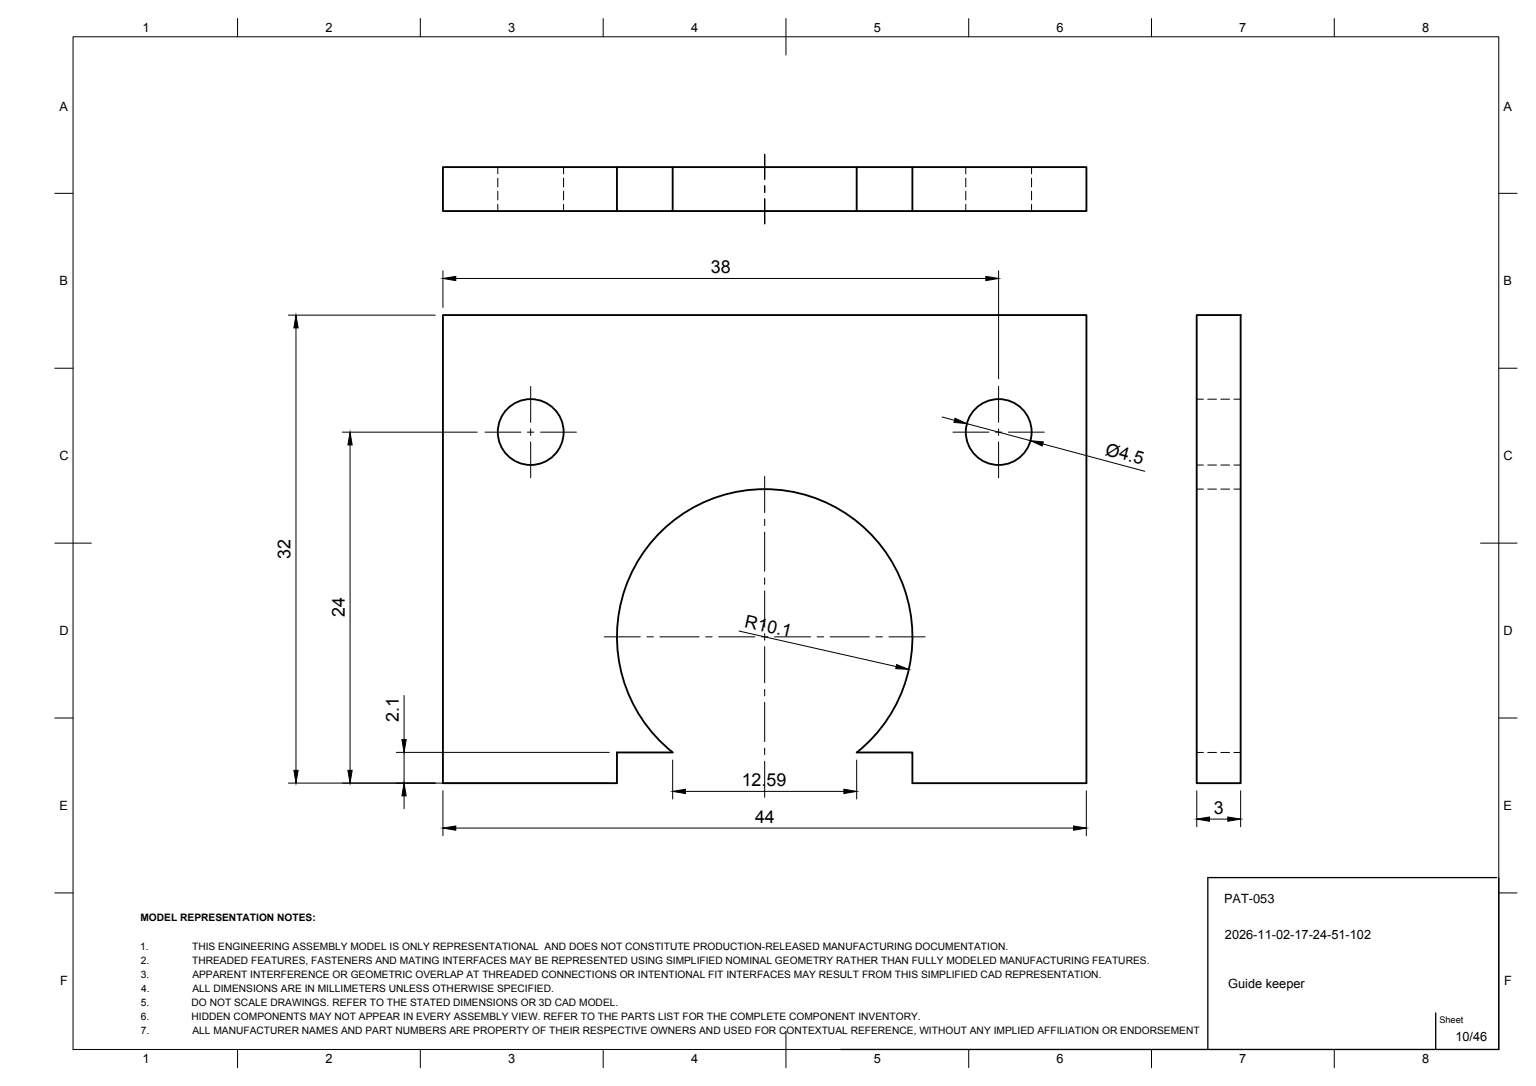
ISO-10303-21;
HEADER;
/* Generated by software containing ST-Developer
 * from STEP Tools, Inc. (www.steptools.com) 
 */

FILE_DESCRIPTION(
/* description */ ('Hand-operated arbor press'),
/* implementation_level */ '2;1');

FILE_NAME(
/* name */ 'Guide keeper.step',
/* time_stamp */ '2026-10-28T03:25:25-07:00',
/* author */ (''),
/* organization */ (''),
/* preprocessor_version */ 'ST-DEVELOPER v20.2',
/* originating_system */ 'Autodesk Translation Framework v15.17.0.0',
/* authorisation */ '');

FILE_SCHEMA (('AUTOMOTIVE_DESIGN { 1 0 10303 214 3 1 1 }'));
ENDSEC;

DATA;
#10=MECHANICAL_DESIGN_GEOMETRIC_PRESENTATION_REPRESENTATION('',(#591),#32751);
#507=SHAPE_REPRESENTATION_RELATIONSHIP('SRR','None',#32936,#549);
#549=ADVANCED_BREP_SHAPE_REPRESENTATION('',(#640),#32710);
#591=STYLED_ITEM('',(#33235),#640);
#640=MANIFOLD_SOLID_BREP('Body1',#12488);
#715=FACE_BOUND('',#2097,.T.);
#716=FACE_BOUND('',#2098,.T.);
#717=FACE_BOUND('',#2104,.T.);
#718=FACE_BOUND('',#2105,.T.);
#901=PLANE('',#13146);
#902=PLANE('',#13147);
#903=PLANE('',#13148);
#904=PLANE('',#13149);
#905=PLANE('',#13150);
#906=PLANE('',#13151);
#907=PLANE('',#13152);
#908=PLANE('',#13156);
#909=PLANE('',#13157);
#910=PLANE('',#13158);
#911=PLANE('',#13159);
#1372=FACE_OUTER_BOUND('',#2088,.T.);
#1373=FACE_OUTER_BOUND('',#2089,.T.);
#1374=FACE_OUTER_BOUND('',#2090,.T.);
#1375=FACE_OUTER_BOUND('',#2091,.T.);
#1376=FACE_OUTER_BOUND('',#2092,.T.);
#1377=FACE_OUTER_BOUND('',#2093,.T.);
#1378=FACE_OUTER_BOUND('',#2094,.T.);
#1379=FACE_OUTER_BOUND('',#2095,.T.);
#1380=FACE_OUTER_BOUND('',#2096,.T.);
#1381=FACE_OUTER_BOUND('',#2099,.T.);
#1382=FACE_OUTER_BOUND('',#2100,.T.);
#1383=FACE_OUTER_BOUND('',#2101,.T.);
#1384=FACE_OUTER_BOUND('',#2102,.T.);
#1385=FACE_OUTER_BOUND('',#2103,.T.);
#2088=EDGE_LOOP('',(#8696,#8697,#8698,#8699));
#2089=EDGE_LOOP('',(#8700,#8701,#8702,#8703));
#2090=EDGE_LOOP('',(#8704,#8705,#8706,#8707));
#2091=EDGE_LOOP('',(#8708,#8709,#8710,#8711));
#2092=EDGE_LOOP('',(#8712,#8713,#8714,#8715));
#2093=EDGE_LOOP('',(#8716,#8717,#8718,#8719));
#2094=EDGE_LOOP('',(#8720,#8721,#8722,#8723));
#2095=EDGE_LOOP('',(#8724,#8725,#8726,#8727));
#2096=EDGE_LOOP('',(#8728,#8729,#8730,#8731,#8732,#8733,#8734,#8735,#8736,
#8737));
#2097=EDGE_LOOP('',(#8738));
#2098=EDGE_LOOP('',(#8739));
#2099=EDGE_LOOP('',(#8740,#8741,#8742,#8743));
#2100=EDGE_LOOP('',(#8744,#8745,#8746,#8747));
#2101=EDGE_LOOP('',(#8748,#8749,#8750,#8751));
#2102=EDGE_LOOP('',(#8752,#8753,#8754,#8755));
#2103=EDGE_LOOP('',(#8756,#8757,#8758,#8759,#8760,#8761,#8762,#8763,#8764,
#8765));
#2104=EDGE_LOOP('',(#8766));
#2105=EDGE_LOOP('',(#8767));
#2956=LINE('',#18039,#4127);
#2957=LINE('',#18045,#4128);
#2958=LINE('',#18050,#4129);
#2959=LINE('',#18052,#4130);
#2960=LINE('',#18054,#4131);
#2961=LINE('',#18055,#4132);
#2962=LINE('',#18059,#4133);
#2963=LINE('',#18061,#4134);
#2964=LINE('',#18063,#4135);
#2965=LINE('',#18064,#4136);
#2966=LINE('',#18067,#4137);
#2967=LINE('',#18069,#4138);
#2968=LINE('',#18070,#4139);
#2969=LINE('',#18073,#4140);
#2970=LINE('',#18075,#4141);
#2971=LINE('',#18076,#4142);
#2972=LINE('',#18079,#4143);
#2973=LINE('',#18081,#4144);
#2974=LINE('',#18082,#4145);
#2975=LINE('',#18085,#4146);
#2976=LINE('',#18087,#4147);
#2977=LINE('',#18088,#4148);
#2978=LINE('',#18092,#4149);
#2979=LINE('',#18094,#4150);
#2980=LINE('',#18095,#4151);
#2981=LINE('',#18100,#4152);
#2982=LINE('',#18101,#4153);
#2983=LINE('',#18104,#4154);
#2984=LINE('',#18105,#4155);
#2985=LINE('',#18107,#4156);
#4127=VECTOR('',#14573,0.225);
#4128=VECTOR('',#14580,0.225);
#4129=VECTOR('',#14585,1.);
#4130=VECTOR('',#14586,1.);
#4131=VECTOR('',#14587,1.);
#4132=VECTOR('',#14588,1.);
#4133=VECTOR('',#14591,1.);
#4134=VECTOR('',#14592,1.);
#4135=VECTOR('',#14593,1.);
#4136=VECTOR('',#14594,1.);
#4137=VECTOR('',#14597,1.);
#4138=VECTOR('',#14598,1.);
#4139=VECTOR('',#14599,1.);
#4140=VECTOR('',#14602,1.);
#4141=VECTOR('',#14603,1.);
#4142=VECTOR('',#14604,1.);
#4143=VECTOR('',#14607,1.);
#4144=VECTOR('',#14608,1.);
#4145=VECTOR('',#14609,1.);
#4146=VECTOR('',#14612,1.);
#4147=VECTOR('',#14613,1.);
#4148=VECTOR('',#14614,1.);
#4149=VECTOR('',#14619,1.);
#4150=VECTOR('',#14620,1.);
#4151=VECTOR('',#14621,1.);
#4152=VECTOR('',#14628,1.);
#4153=VECTOR('',#14629,1.);
#4154=VECTOR('',#14632,1.);
#4155=VECTOR('',#14633,1.);
#4156=VECTOR('',#14636,1.);
#5220=CIRCLE('',#13141,0.225);
#5221=CIRCLE('',#13142,0.225);
#5222=CIRCLE('',#13144,0.225);
#5223=CIRCLE('',#13145,0.225);
#5224=CIRCLE('',#13153,1.01);
#5225=CIRCLE('',#13155,1.01);
#5680=VERTEX_POINT('',#18036);
#5681=VERTEX_POINT('',#18038);
#5682=VERTEX_POINT('',#18042);
#5683=VERTEX_POINT('',#18044);
#5684=VERTEX_POINT('',#18048);
#5685=VERTEX_POINT('',#18049);
#5686=VERTEX_POINT('',#18051);
#5687=VERTEX_POINT('',#18053);
#5688=VERTEX_POINT('',#18057);
#5689=VERTEX_POINT('',#18058);
#5690=VERTEX_POINT('',#18060);
#5691=VERTEX_POINT('',#18062);
#5692=VERTEX_POINT('',#18066);
#5693=VERTEX_POINT('',#18068);
#5694=VERTEX_POINT('',#18072);
#5695=VERTEX_POINT('',#18074);
#5696=VERTEX_POINT('',#18078);
#5697=VERTEX_POINT('',#18080);
#5698=VERTEX_POINT('',#18084);
#5699=VERTEX_POINT('',#18086);
#5700=VERTEX_POINT('',#18091);
#5701=VERTEX_POINT('',#18093);
#5702=VERTEX_POINT('',#18099);
#5703=VERTEX_POINT('',#18103);
#6851=EDGE_CURVE('',#5680,#5680,#5220,.T.);
#6852=EDGE_CURVE('',#5680,#5681,#2956,.T.);
#6853=EDGE_CURVE('',#5681,#5681,#5221,.T.);
#6854=EDGE_CURVE('',#5682,#5682,#5222,.T.);
#6855=EDGE_CURVE('',#5682,#5683,#2957,.T.);
#6856=EDGE_CURVE('',#5683,#5683,#5223,.T.);
#6857=EDGE_CURVE('',#5684,#5685,#2958,.T.);
#6858=EDGE_CURVE('',#5684,#5686,#2959,.T.);
#6859=EDGE_CURVE('',#5687,#5686,#2960,.T.);
#6860=EDGE_CURVE('',#5685,#5687,#2961,.T.);
#6861=EDGE_CURVE('',#5688,#5689,#2962,.T.);
#6862=EDGE_CURVE('',#5690,#5688,#2963,.T.);
#6863=EDGE_CURVE('',#5691,#5690,#2964,.T.);
#6864=EDGE_CURVE('',#5689,#5691,#2965,.T.);
#6865=EDGE_CURVE('',#5692,#5688,#2966,.T.);
#6866=EDGE_CURVE('',#5693,#5692,#2967,.T.);
#6867=EDGE_CURVE('',#5690,#5693,#2968,.T.);
#6868=EDGE_CURVE('',#5694,#5684,#2969,.T.);
#6869=EDGE_CURVE('',#5695,#5694,#2970,.T.);
#6870=EDGE_CURVE('',#5686,#5695,#2971,.T.);
#6871=EDGE_CURVE('',#5696,#5687,#2972,.T.);
#6872=EDGE_CURVE('',#5697,#5696,#2973,.T.);
#6873=EDGE_CURVE('',#5697,#5685,#2974,.T.);
#6874=EDGE_CURVE('',#5691,#5698,#2975,.T.);
#6875=EDGE_CURVE('',#5698,#5699,#2976,.T.);
#6876=EDGE_CURVE('',#5689,#5699,#2977,.T.);
#6877=EDGE_CURVE('',#5695,#5692,#5224,.T.);
#6878=EDGE_CURVE('',#5699,#5700,#2978,.T.);
#6879=EDGE_CURVE('',#5700,#5701,#2979,.T.);
#6880=EDGE_CURVE('',#5701,#5696,#2980,.T.);
#6881=EDGE_CURVE('',#5693,#5694,#5225,.T.);
#6882=EDGE_CURVE('',#5702,#5697,#2981,.T.);
#6883=EDGE_CURVE('',#5702,#5701,#2982,.T.);
#6884=EDGE_CURVE('',#5703,#5702,#2983,.T.);
#6885=EDGE_CURVE('',#5703,#5700,#2984,.T.);
#6886=EDGE_CURVE('',#5698,#5703,#2985,.T.);
#8696=ORIENTED_EDGE('',*,*,#6851,.F.);
#8697=ORIENTED_EDGE('',*,*,#6852,.T.);
#8698=ORIENTED_EDGE('',*,*,#6853,.F.);
#8699=ORIENTED_EDGE('',*,*,#6852,.F.);
#8700=ORIENTED_EDGE('',*,*,#6854,.F.);
#8701=ORIENTED_EDGE('',*,*,#6855,.T.);
#8702=ORIENTED_EDGE('',*,*,#6856,.F.);
#8703=ORIENTED_EDGE('',*,*,#6855,.F.);
#8704=ORIENTED_EDGE('',*,*,#6857,.F.);
#8705=ORIENTED_EDGE('',*,*,#6858,.T.);
#8706=ORIENTED_EDGE('',*,*,#6859,.F.);
#8707=ORIENTED_EDGE('',*,*,#6860,.F.);
#8708=ORIENTED_EDGE('',*,*,#6861,.F.);
#8709=ORIENTED_EDGE('',*,*,#6862,.F.);
#8710=ORIENTED_EDGE('',*,*,#6863,.F.);
#8711=ORIENTED_EDGE('',*,*,#6864,.F.);
#8712=ORIENTED_EDGE('',*,*,#6865,.F.);
#8713=ORIENTED_EDGE('',*,*,#6866,.F.);
#8714=ORIENTED_EDGE('',*,*,#6867,.F.);
#8715=ORIENTED_EDGE('',*,*,#6862,.T.);
#8716=ORIENTED_EDGE('',*,*,#6868,.F.);
#8717=ORIENTED_EDGE('',*,*,#6869,.F.);
#8718=ORIENTED_EDGE('',*,*,#6870,.F.);
#8719=ORIENTED_EDGE('',*,*,#6858,.F.);
#8720=ORIENTED_EDGE('',*,*,#6860,.T.);
#8721=ORIENTED_EDGE('',*,*,#6871,.F.);
#8722=ORIENTED_EDGE('',*,*,#6872,.F.);
#8723=ORIENTED_EDGE('',*,*,#6873,.T.);
#8724=ORIENTED_EDGE('',*,*,#6864,.T.);
#8725=ORIENTED_EDGE('',*,*,#6874,.T.);
#8726=ORIENTED_EDGE('',*,*,#6875,.T.);
#8727=ORIENTED_EDGE('',*,*,#6876,.F.);
#8728=ORIENTED_EDGE('',*,*,#6859,.T.);
#8729=ORIENTED_EDGE('',*,*,#6870,.T.);
#8730=ORIENTED_EDGE('',*,*,#6877,.T.);
#8731=ORIENTED_EDGE('',*,*,#6865,.T.);
#8732=ORIENTED_EDGE('',*,*,#6861,.T.);
#8733=ORIENTED_EDGE('',*,*,#6876,.T.);
#8734=ORIENTED_EDGE('',*,*,#6878,.T.);
#8735=ORIENTED_EDGE('',*,*,#6879,.T.);
#8736=ORIENTED_EDGE('',*,*,#6880,.T.);
#8737=ORIENTED_EDGE('',*,*,#6871,.T.);
#8738=ORIENTED_EDGE('',*,*,#6853,.T.);
#8739=ORIENTED_EDGE('',*,*,#6856,.T.);
#8740=ORIENTED_EDGE('',*,*,#6869,.T.);
#8741=ORIENTED_EDGE('',*,*,#6881,.F.);
#8742=ORIENTED_EDGE('',*,*,#6866,.T.);
#8743=ORIENTED_EDGE('',*,*,#6877,.F.);
#8744=ORIENTED_EDGE('',*,*,#6882,.T.);
#8745=ORIENTED_EDGE('',*,*,#6872,.T.);
#8746=ORIENTED_EDGE('',*,*,#6880,.F.);
#8747=ORIENTED_EDGE('',*,*,#6883,.F.);
#8748=ORIENTED_EDGE('',*,*,#6884,.T.);
#8749=ORIENTED_EDGE('',*,*,#6883,.T.);
#8750=ORIENTED_EDGE('',*,*,#6879,.F.);
#8751=ORIENTED_EDGE('',*,*,#6885,.F.);
#8752=ORIENTED_EDGE('',*,*,#6886,.T.);
#8753=ORIENTED_EDGE('',*,*,#6885,.T.);
#8754=ORIENTED_EDGE('',*,*,#6878,.F.);
#8755=ORIENTED_EDGE('',*,*,#6875,.F.);
#8756=ORIENTED_EDGE('',*,*,#6857,.T.);
#8757=ORIENTED_EDGE('',*,*,#6873,.F.);
#8758=ORIENTED_EDGE('',*,*,#6882,.F.);
#8759=ORIENTED_EDGE('',*,*,#6884,.F.);
#8760=ORIENTED_EDGE('',*,*,#6886,.F.);
#8761=ORIENTED_EDGE('',*,*,#6874,.F.);
#8762=ORIENTED_EDGE('',*,*,#6863,.T.);
#8763=ORIENTED_EDGE('',*,*,#6867,.T.);
#8764=ORIENTED_EDGE('',*,*,#6881,.T.);
#8765=ORIENTED_EDGE('',*,*,#6868,.T.);
#8766=ORIENTED_EDGE('',*,*,#6851,.T.);
#8767=ORIENTED_EDGE('',*,*,#6854,.T.);
#11669=CYLINDRICAL_SURFACE('',#13140,0.225);
#11670=CYLINDRICAL_SURFACE('',#13143,0.225);
#11671=CYLINDRICAL_SURFACE('',#13154,1.01);
#11881=ADVANCED_FACE('',(#1372),#11669,.F.);
#11882=ADVANCED_FACE('',(#1373),#11670,.F.);
#11883=ADVANCED_FACE('',(#1374),#901,.F.);
#11884=ADVANCED_FACE('',(#1375),#902,.F.);
#11885=ADVANCED_FACE('',(#1376),#903,.F.);
#11886=ADVANCED_FACE('',(#1377),#904,.F.);
#11887=ADVANCED_FACE('',(#1378),#905,.T.);
#11888=ADVANCED_FACE('',(#1379),#906,.T.);
#11889=ADVANCED_FACE('',(#1380,#715,#716),#907,.T.);
#11890=ADVANCED_FACE('',(#1381),#11671,.F.);
#11891=ADVANCED_FACE('',(#1382),#908,.T.);
#11892=ADVANCED_FACE('',(#1383),#909,.T.);
#11893=ADVANCED_FACE('',(#1384),#910,.T.);
#11894=ADVANCED_FACE('',(#1385,#717,#718),#911,.F.);
#12488=CLOSED_SHELL('',(#11881,#11882,#11883,#11884,#11885,#11886,#11887,
#11888,#11889,#11890,#11891,#11892,#11893,#11894));
#13139=AXIS2_PLACEMENT_3D('',#18034,#14567,#14568);
#13140=AXIS2_PLACEMENT_3D('',#18035,#14569,#14570);
#13141=AXIS2_PLACEMENT_3D('',#18037,#14571,#14572);
#13142=AXIS2_PLACEMENT_3D('',#18040,#14574,#14575);
#13143=AXIS2_PLACEMENT_3D('',#18041,#14576,#14577);
#13144=AXIS2_PLACEMENT_3D('',#18043,#14578,#14579);
#13145=AXIS2_PLACEMENT_3D('',#18046,#14581,#14582);
#13146=AXIS2_PLACEMENT_3D('',#18047,#14583,#14584);
#13147=AXIS2_PLACEMENT_3D('',#18056,#14589,#14590);
#13148=AXIS2_PLACEMENT_3D('',#18065,#14595,#14596);
#13149=AXIS2_PLACEMENT_3D('',#18071,#14600,#14601);
#13150=AXIS2_PLACEMENT_3D('',#18077,#14605,#14606);
#13151=AXIS2_PLACEMENT_3D('',#18083,#14610,#14611);
#13152=AXIS2_PLACEMENT_3D('',#18089,#14615,#14616);
#13153=AXIS2_PLACEMENT_3D('',#18090,#14617,#14618);
#13154=AXIS2_PLACEMENT_3D('',#18096,#14622,#14623);
#13155=AXIS2_PLACEMENT_3D('',#18097,#14624,#14625);
#13156=AXIS2_PLACEMENT_3D('',#18098,#14626,#14627);
#13157=AXIS2_PLACEMENT_3D('',#18102,#14630,#14631);
#13158=AXIS2_PLACEMENT_3D('',#18106,#14634,#14635);
#13159=AXIS2_PLACEMENT_3D('',#18108,#14637,#14638);
#14567=DIRECTION('axis',(0.,0.,1.));
#14568=DIRECTION('refdir',(1.,0.,0.));
#14569=DIRECTION('center_axis',(0.,0.,1.));
#14570=DIRECTION('ref_axis',(1.,0.,0.));
#14571=DIRECTION('center_axis',(0.,0.,1.));
#14572=DIRECTION('ref_axis',(1.,0.,0.));
#14573=DIRECTION('',(0.,0.,1.));
#14574=DIRECTION('center_axis',(0.,0.,-1.));
#14575=DIRECTION('ref_axis',(1.,0.,0.));
#14576=DIRECTION('center_axis',(0.,0.,1.));
#14577=DIRECTION('ref_axis',(1.,0.,0.));
#14578=DIRECTION('center_axis',(0.,0.,1.));
#14579=DIRECTION('ref_axis',(1.,0.,0.));
#14580=DIRECTION('',(0.,0.,1.));
#14581=DIRECTION('center_axis',(0.,0.,-1.));
#14582=DIRECTION('ref_axis',(1.,0.,0.));
#14583=DIRECTION('center_axis',(0.,1.,0.));
#14584=DIRECTION('ref_axis',(-1.,0.,0.));
#14585=DIRECTION('',(-1.,0.,0.));
#14586=DIRECTION('',(0.,0.,1.));
#14587=DIRECTION('',(1.,0.,0.));
#14588=DIRECTION('',(0.,0.,1.));
#14589=DIRECTION('center_axis',(0.,-1.,0.));
#14590=DIRECTION('ref_axis',(1.,0.,0.));
#14591=DIRECTION('',(-1.,0.,0.));
#14592=DIRECTION('',(0.,0.,1.));
#14593=DIRECTION('',(1.,0.,0.));
#14594=DIRECTION('',(0.,0.,-1.));
#14595=DIRECTION('center_axis',(1.,0.,0.));
#14596=DIRECTION('ref_axis',(0.,1.,0.));
#14597=DIRECTION('',(0.,-1.,0.));
#14598=DIRECTION('',(0.,0.,1.));
#14599=DIRECTION('',(0.,1.,0.));
#14600=DIRECTION('center_axis',(1.,0.,0.));
#14601=DIRECTION('ref_axis',(0.,1.,0.));
#14602=DIRECTION('',(0.,1.,0.));
#14603=DIRECTION('',(0.,0.,-1.));
#14604=DIRECTION('',(0.,-1.,0.));
#14605=DIRECTION('center_axis',(-1.,0.,0.));
#14606=DIRECTION('ref_axis',(0.,-1.,0.));
#14607=DIRECTION('',(0.,-1.,0.));
#14608=DIRECTION('',(0.,0.,1.));
#14609=DIRECTION('',(0.,-1.,0.));
#14610=DIRECTION('center_axis',(-1.,0.,0.));
#14611=DIRECTION('ref_axis',(0.,-1.,0.));
#14612=DIRECTION('',(0.,-1.,0.));
#14613=DIRECTION('',(0.,0.,1.));
#14614=DIRECTION('',(0.,-1.,0.));
#14615=DIRECTION('center_axis',(0.,0.,1.));
#14616=DIRECTION('ref_axis',(1.,0.,0.));
#14617=DIRECTION('center_axis',(0.,0.,-1.));
#14618=DIRECTION('ref_axis',(1.,0.,0.));
#14619=DIRECTION('',(1.,0.,0.));
#14620=DIRECTION('',(0.,1.,0.));
#14621=DIRECTION('',(-1.,0.,0.));
#14622=DIRECTION('center_axis',(0.,0.,1.));
#14623=DIRECTION('ref_axis',(1.,0.,0.));
#14624=DIRECTION('center_axis',(0.,0.,1.));
#14625=DIRECTION('ref_axis',(1.,0.,0.));
#14626=DIRECTION('center_axis',(0.,1.,0.));
#14627=DIRECTION('ref_axis',(-1.,0.,0.));
#14628=DIRECTION('',(-1.,0.,0.));
#14629=DIRECTION('',(0.,0.,1.));
#14630=DIRECTION('center_axis',(1.,0.,0.));
#14631=DIRECTION('ref_axis',(0.,1.,0.));
#14632=DIRECTION('',(0.,1.,0.));
#14633=DIRECTION('',(0.,0.,1.));
#14634=DIRECTION('center_axis',(0.,-1.,0.));
#14635=DIRECTION('ref_axis',(1.,0.,0.));
#14636=DIRECTION('',(1.,0.,0.));
#14637=DIRECTION('center_axis',(0.,0.,1.));
#14638=DIRECTION('ref_axis',(1.,0.,0.));
#18034=CARTESIAN_POINT('',(0.,0.,0.));
#18035=CARTESIAN_POINT('Origin',(2.4,-1.6,15.2));
#18036=CARTESIAN_POINT('',(2.175,-1.6,15.3));
#18037=CARTESIAN_POINT('Origin',(2.4,-1.6,15.3));
#18038=CARTESIAN_POINT('',(2.175,-1.6,15.6));
#18039=CARTESIAN_POINT('',(2.175,-1.6,15.2));
#18040=CARTESIAN_POINT('Origin',(2.4,-1.6,15.6));
#18041=CARTESIAN_POINT('Origin',(2.4,1.6,15.2));
#18042=CARTESIAN_POINT('',(2.175,1.6,15.3));
#18043=CARTESIAN_POINT('Origin',(2.4,1.6,15.3));
#18044=CARTESIAN_POINT('',(2.175,1.6,15.6));
#18045=CARTESIAN_POINT('',(2.175,1.6,15.2));
#18046=CARTESIAN_POINT('Origin',(2.4,1.6,15.6));
#18047=CARTESIAN_POINT('Origin',(0.21,1.01,15.2));
#18048=CARTESIAN_POINT('',(0.21,1.01,15.3));
#18049=CARTESIAN_POINT('',(0.,1.01,15.3));
#18050=CARTESIAN_POINT('',(0.905,1.01,15.3));
#18051=CARTESIAN_POINT('',(0.21,1.01,15.6));
#18052=CARTESIAN_POINT('',(0.21,1.01,15.2));
#18053=CARTESIAN_POINT('',(0.,1.01,15.6));
#18054=CARTESIAN_POINT('',(0.905,1.01,15.6));
#18055=CARTESIAN_POINT('',(0.,1.01,15.25));
#18056=CARTESIAN_POINT('Origin',(-0.1,-1.01,15.2));
#18057=CARTESIAN_POINT('',(0.21,-1.01,15.6));
#18058=CARTESIAN_POINT('',(0.,-1.01,15.6));
#18059=CARTESIAN_POINT('',(0.75,-1.01,15.6));
#18060=CARTESIAN_POINT('',(0.21,-1.01,15.3));
#18061=CARTESIAN_POINT('',(0.21,-1.01,15.2));
#18062=CARTESIAN_POINT('',(0.,-1.01,15.3));
#18063=CARTESIAN_POINT('',(0.75,-1.01,15.3));
#18064=CARTESIAN_POINT('',(0.,-1.01,15.25));
#18065=CARTESIAN_POINT('Origin',(0.21,-1.01,15.2));
#18066=CARTESIAN_POINT('',(0.21,-0.629285308902091,15.6));
#18067=CARTESIAN_POINT('',(0.21,-0.505,15.6));
#18068=CARTESIAN_POINT('',(0.21,-0.629285308902091,15.3));
#18069=CARTESIAN_POINT('',(0.21,-0.629285308902091,15.2));
#18070=CARTESIAN_POINT('',(0.21,-0.505,15.3));
#18071=CARTESIAN_POINT('Origin',(0.21,-1.01,15.2));
#18072=CARTESIAN_POINT('',(0.21,0.629285308902091,15.3));
#18073=CARTESIAN_POINT('',(0.21,-0.505,15.3));
#18074=CARTESIAN_POINT('',(0.21,0.629285308902091,15.6));
#18075=CARTESIAN_POINT('',(0.21,0.629285308902091,15.2));
#18076=CARTESIAN_POINT('',(0.21,-0.505,15.6));
#18077=CARTESIAN_POINT('Origin',(0.,2.2,15.3));
#18078=CARTESIAN_POINT('',(0.,2.2,15.6));
#18079=CARTESIAN_POINT('',(0.,2.2,15.6));
#18080=CARTESIAN_POINT('',(0.,2.2,15.3));
#18081=CARTESIAN_POINT('',(0.,2.2,15.3));
#18082=CARTESIAN_POINT('',(0.,2.2,15.3));
#18083=CARTESIAN_POINT('Origin',(0.,2.2,15.3));
#18084=CARTESIAN_POINT('',(0.,-2.2,15.3));
#18085=CARTESIAN_POINT('',(0.,2.2,15.3));
#18086=CARTESIAN_POINT('',(0.,-2.2,15.6));
#18087=CARTESIAN_POINT('',(0.,-2.2,15.3));
#18088=CARTESIAN_POINT('',(0.,2.2,15.6));
#18089=CARTESIAN_POINT('Origin',(1.6,0.,15.6));
#18090=CARTESIAN_POINT('Origin',(1.,0.,15.6));
#18091=CARTESIAN_POINT('',(3.2,-2.2,15.6));
#18092=CARTESIAN_POINT('',(0.,-2.2,15.6));
#18093=CARTESIAN_POINT('',(3.2,2.2,15.6));
#18094=CARTESIAN_POINT('',(3.2,-2.2,15.6));
#18095=CARTESIAN_POINT('',(3.2,2.2,15.6));
#18096=CARTESIAN_POINT('Origin',(1.,0.,15.2));
#18097=CARTESIAN_POINT('Origin',(1.,0.,15.3));
#18098=CARTESIAN_POINT('Origin',(3.2,2.2,15.3));
#18099=CARTESIAN_POINT('',(3.2,2.2,15.3));
#18100=CARTESIAN_POINT('',(3.2,2.2,15.3));
#18101=CARTESIAN_POINT('',(3.2,2.2,15.3));
#18102=CARTESIAN_POINT('Origin',(3.2,-2.2,15.3));
#18103=CARTESIAN_POINT('',(3.2,-2.2,15.3));
#18104=CARTESIAN_POINT('',(3.2,-2.2,15.3));
#18105=CARTESIAN_POINT('',(3.2,-2.2,15.3));
#18106=CARTESIAN_POINT('Origin',(0.,-2.2,15.3));
#18107=CARTESIAN_POINT('',(0.,-2.2,15.3));
#18108=CARTESIAN_POINT('Origin',(1.6,0.,15.3));
#32661=UNCERTAINTY_MEASURE_WITH_UNIT(LENGTH_MEASURE(0.001),#32752,
'DISTANCE_ACCURACY_VALUE',
'Maximum model space distance between geometric entities at asserted c
onnectivities');
#32702=UNCERTAINTY_MEASURE_WITH_UNIT(LENGTH_MEASURE(0.001),#32752,
'DISTANCE_ACCURACY_VALUE',
'Maximum model space distance between geometric entities at asserted c
onnectivities');
#32710=(
GEOMETRIC_REPRESENTATION_CONTEXT(3)
GLOBAL_UNCERTAINTY_ASSIGNED_CONTEXT((#32661))
GLOBAL_UNIT_ASSIGNED_CONTEXT((#32752,#32754,#32755))
REPRESENTATION_CONTEXT('','3D')
);
#32751=(
GEOMETRIC_REPRESENTATION_CONTEXT(3)
GLOBAL_UNCERTAINTY_ASSIGNED_CONTEXT((#32702))
GLOBAL_UNIT_ASSIGNED_CONTEXT((#32752,#32754,#32755))
REPRESENTATION_CONTEXT('','3D')
);
#32752=(
LENGTH_UNIT()
NAMED_UNIT(*)
SI_UNIT(.CENTI.,.METRE.)
);
#32754=(
NAMED_UNIT(*)
PLANE_ANGLE_UNIT()
SI_UNIT($,.RADIAN.)
);
#32755=(
NAMED_UNIT(*)
SI_UNIT($,.STERADIAN.)
SOLID_ANGLE_UNIT()
);
#32763=SHAPE_DEFINITION_REPRESENTATION(#32811,#32936);
#32811=PRODUCT_DEFINITION_SHAPE('',$,#32985);
#32936=SHAPE_REPRESENTATION('',(#13139),#32710);
#32977=PRODUCT_DEFINITION_CONTEXT('part definition',#33123,'design');
#32985=PRODUCT_DEFINITION('Guide keeper','Guide keeper',#33033,#32977);
#33033=PRODUCT_DEFINITION_FORMATION('',$,#33132);
#33123=APPLICATION_CONTEXT(
'Core Data for Automotive Mechanical Design Process');
#33124=PRODUCT_CONTEXT('part definition',#33123,'mechanical');
#33132=PRODUCT('Guide keeper','Guide keeper','Guide keeper',(#33124));
#33229=COLOUR_RGB('Sky Blue',0.24,0.69,0.87);
#33230=FILL_AREA_STYLE_COLOUR('',#33229);
#33231=FILL_AREA_STYLE('',(#33230));
#33232=SURFACE_STYLE_FILL_AREA(#33231);
#33233=SURFACE_SIDE_STYLE('',(#33232));
#33234=SURFACE_STYLE_USAGE(.BOTH.,#33233);
#33235=PRESENTATION_STYLE_ASSIGNMENT((#33234));
ENDSEC;
END-ISO-10303-21;
